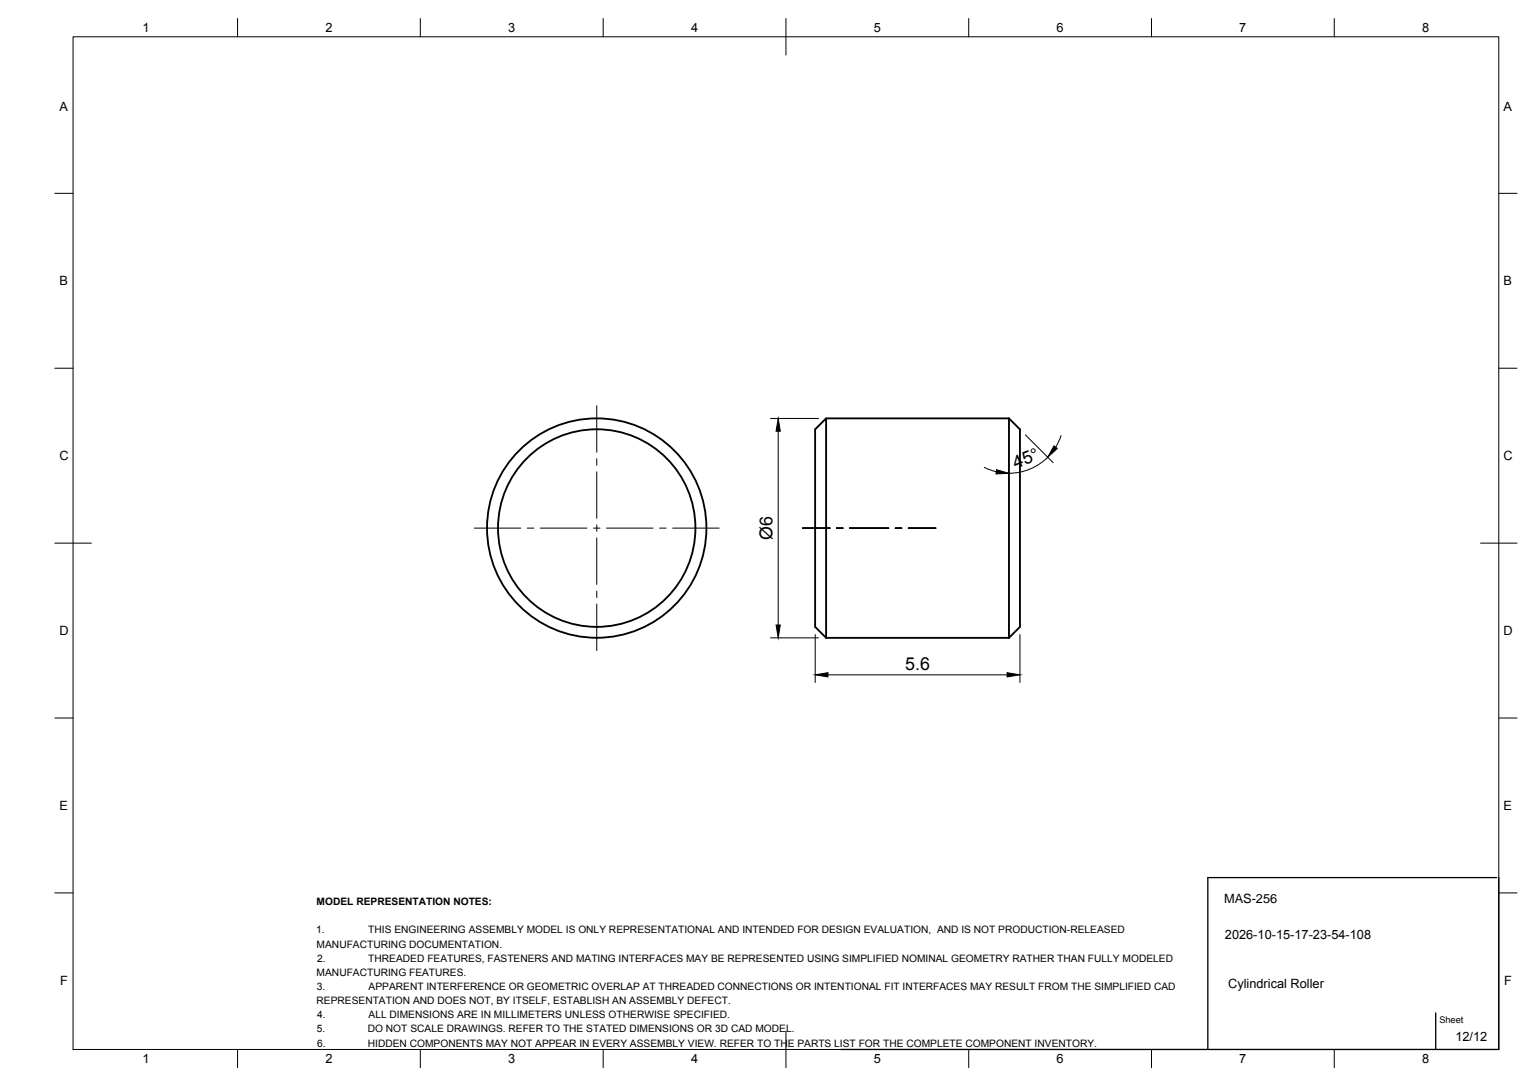
ISO-10303-21;
HEADER;
/* Generated by software containing ST-Developer
 * from STEP Tools, Inc. (www.steptools.com) 
 */

FILE_DESCRIPTION(
/* description */ (''),
/* implementation_level */ '2;1');

FILE_NAME(
/* name */ 'Cylindrical Roller.step',
/* time_stamp */ '2026-10-14T18:40:07-07:00',
/* author */ (''),
/* organization */ (''),
/* preprocessor_version */ 'ST-DEVELOPER v20.2',
/* originating_system */ 'Autodesk Translation Framework v15.15.0.0',
/* authorisation */ '');

FILE_SCHEMA (('AUTOMOTIVE_DESIGN { 1 0 10303 214 3 1 1 }'));
ENDSEC;

DATA;
#10=MECHANICAL_DESIGN_GEOMETRIC_PRESENTATION_REPRESENTATION('',(#836),#81040);
#816=SHAPE_REPRESENTATION_RELATIONSHIP('SRR','None',#81135,#826);
#826=ADVANCED_BREP_SHAPE_REPRESENTATION('',(#846),#81035);
#836=STYLED_ITEM('',(#81194),#846);
#846=MANIFOLD_SOLID_BREP('Body1',#15089);
#990=CYLINDRICAL_SURFACE('',#16080,3.);
#1428=PLANE('',#16076);
#1429=PLANE('',#16084);
#2049=FACE_OUTER_BOUND('',#2915,.T.);
#2050=FACE_OUTER_BOUND('',#2916,.T.);
#2051=FACE_OUTER_BOUND('',#2917,.T.);
#2052=FACE_OUTER_BOUND('',#2918,.T.);
#2053=FACE_OUTER_BOUND('',#2919,.T.);
#2915=EDGE_LOOP('',(#12168));
#2916=EDGE_LOOP('',(#12169,#12170,#12171,#12172));
#2917=EDGE_LOOP('',(#12173,#12174,#12175,#12176));
#2918=EDGE_LOOP('',(#12177,#12178,#12179,#12180));
#2919=EDGE_LOOP('',(#12181));
#3986=LINE('',#23024,#5098);
#3987=LINE('',#23028,#5099);
#3988=LINE('',#23031,#5100);
#5098=VECTOR('',#19136,2.85);
#5099=VECTOR('',#19141,3.);
#5100=VECTOR('',#19144,2.85);
#5837=CIRCLE('',#16077,2.7);
#5838=CIRCLE('',#16079,3.);
#5839=CIRCLE('',#16081,3.);
#5840=CIRCLE('',#16083,2.7);
#6804=VERTEX_POINT('',#23019);
#6805=VERTEX_POINT('',#23022);
#6806=VERTEX_POINT('',#23026);
#6807=VERTEX_POINT('',#23030);
#8747=EDGE_CURVE('',#6804,#6804,#5837,.T.);
#8748=EDGE_CURVE('',#6805,#6805,#5838,.T.);
#8749=EDGE_CURVE('',#6805,#6804,#3986,.T.);
#8750=EDGE_CURVE('',#6806,#6806,#5839,.T.);
#8751=EDGE_CURVE('',#6806,#6805,#3987,.T.);
#8752=EDGE_CURVE('',#6806,#6807,#3988,.T.);
#8753=EDGE_CURVE('',#6807,#6807,#5840,.T.);
#12168=ORIENTED_EDGE('',*,*,#8747,.F.);
#12169=ORIENTED_EDGE('',*,*,#8748,.F.);
#12170=ORIENTED_EDGE('',*,*,#8749,.T.);
#12171=ORIENTED_EDGE('',*,*,#8747,.T.);
#12172=ORIENTED_EDGE('',*,*,#8749,.F.);
#12173=ORIENTED_EDGE('',*,*,#8750,.F.);
#12174=ORIENTED_EDGE('',*,*,#8751,.T.);
#12175=ORIENTED_EDGE('',*,*,#8748,.T.);
#12176=ORIENTED_EDGE('',*,*,#8751,.F.);
#12177=ORIENTED_EDGE('',*,*,#8750,.T.);
#12178=ORIENTED_EDGE('',*,*,#8752,.T.);
#12179=ORIENTED_EDGE('',*,*,#8753,.F.);
#12180=ORIENTED_EDGE('',*,*,#8752,.F.);
#12181=ORIENTED_EDGE('',*,*,#8753,.T.);
#14325=CONICAL_SURFACE('',#16078,2.85,0.785398163397441);
#14326=CONICAL_SURFACE('',#16082,2.85,0.785398163397434);
#14784=ADVANCED_FACE('',(#2049),#1428,.T.);
#14785=ADVANCED_FACE('',(#2050),#14325,.T.);
#14786=ADVANCED_FACE('',(#2051),#990,.T.);
#14787=ADVANCED_FACE('',(#2052),#14326,.T.);
#14788=ADVANCED_FACE('',(#2053),#1429,.T.);
#15089=CLOSED_SHELL('',(#14784,#14785,#14786,#14787,#14788));
#16075=AXIS2_PLACEMENT_3D('',#23017,#19126,#19127);
#16076=AXIS2_PLACEMENT_3D('',#23018,#19128,#19129);
#16077=AXIS2_PLACEMENT_3D('',#23020,#19130,#19131);
#16078=AXIS2_PLACEMENT_3D('',#23021,#19132,#19133);
#16079=AXIS2_PLACEMENT_3D('',#23023,#19134,#19135);
#16080=AXIS2_PLACEMENT_3D('',#23025,#19137,#19138);
#16081=AXIS2_PLACEMENT_3D('',#23027,#19139,#19140);
#16082=AXIS2_PLACEMENT_3D('',#23029,#19142,#19143);
#16083=AXIS2_PLACEMENT_3D('',#23032,#19145,#19146);
#16084=AXIS2_PLACEMENT_3D('',#23033,#19147,#19148);
#19126=DIRECTION('axis',(0.,0.,1.));
#19127=DIRECTION('refdir',(1.,0.,0.));
#19128=DIRECTION('center_axis',(0.,1.,0.));
#19129=DIRECTION('ref_axis',(0.,0.,1.));
#19130=DIRECTION('center_axis',(0.,-1.,0.));
#19131=DIRECTION('ref_axis',(1.,0.,0.));
#19132=DIRECTION('center_axis',(0.,-1.,0.));
#19133=DIRECTION('ref_axis',(1.,0.,0.));
#19134=DIRECTION('center_axis',(0.,-1.,0.));
#19135=DIRECTION('ref_axis',(1.,0.,0.));
#19136=DIRECTION('',(0.707106781186542,0.707106781186553,8.65956056235487E-17));
#19137=DIRECTION('center_axis',(0.,-1.,0.));
#19138=DIRECTION('ref_axis',(1.,0.,0.));
#19139=DIRECTION('center_axis',(0.,-1.,0.));
#19140=DIRECTION('ref_axis',(1.,0.,0.));
#19141=DIRECTION('',(0.,1.,0.));
#19142=DIRECTION('center_axis',(0.,1.,0.));
#19143=DIRECTION('ref_axis',(1.,0.,0.));
#19144=DIRECTION('',(0.707106781186537,-0.707106781186558,-8.65956056235481E-17));
#19145=DIRECTION('center_axis',(0.,-1.,0.));
#19146=DIRECTION('ref_axis',(1.,0.,0.));
#19147=DIRECTION('center_axis',(0.,-1.,0.));
#19148=DIRECTION('ref_axis',(0.,0.,-1.));
#23017=CARTESIAN_POINT('',(0.,0.,0.));
#23018=CARTESIAN_POINT('Origin',(47.7,23.8,32.));
#23019=CARTESIAN_POINT('',(42.3,23.8,32.));
#23020=CARTESIAN_POINT('Origin',(45.,23.8,32.));
#23021=CARTESIAN_POINT('Origin',(45.,23.65,32.));
#23022=CARTESIAN_POINT('',(42.,23.5,32.));
#23023=CARTESIAN_POINT('Origin',(45.,23.5,32.));
#23024=CARTESIAN_POINT('',(42.15,23.65,32.));
#23025=CARTESIAN_POINT('Origin',(45.,21.,32.));
#23026=CARTESIAN_POINT('',(42.,18.5,32.));
#23027=CARTESIAN_POINT('Origin',(45.,18.5,32.));
#23028=CARTESIAN_POINT('',(42.,21.,32.));
#23029=CARTESIAN_POINT('Origin',(45.,18.35,32.));
#23030=CARTESIAN_POINT('',(42.3,18.2,32.));
#23031=CARTESIAN_POINT('',(42.15,18.35,32.));
#23032=CARTESIAN_POINT('Origin',(45.,18.2,32.));
#23033=CARTESIAN_POINT('Origin',(45.,18.2,32.));
#81023=UNCERTAINTY_MEASURE_WITH_UNIT(LENGTH_MEASURE(0.01),#81041,
'DISTANCE_ACCURACY_VALUE',
'Maximum model space distance between geometric entities at asserted c
onnectivities');
#81028=UNCERTAINTY_MEASURE_WITH_UNIT(LENGTH_MEASURE(0.01),#81041,
'DISTANCE_ACCURACY_VALUE',
'Maximum model space distance between geometric entities at asserted c
onnectivities');
#81035=(
GEOMETRIC_REPRESENTATION_CONTEXT(3)
GLOBAL_UNCERTAINTY_ASSIGNED_CONTEXT((#81023))
GLOBAL_UNIT_ASSIGNED_CONTEXT((#81041,#81043,#81044))
REPRESENTATION_CONTEXT('','3D')
);
#81040=(
GEOMETRIC_REPRESENTATION_CONTEXT(3)
GLOBAL_UNCERTAINTY_ASSIGNED_CONTEXT((#81028))
GLOBAL_UNIT_ASSIGNED_CONTEXT((#81041,#81043,#81044))
REPRESENTATION_CONTEXT('','3D')
);
#81041=(
LENGTH_UNIT()
NAMED_UNIT(*)
SI_UNIT(.MILLI.,.METRE.)
);
#81043=(
NAMED_UNIT(*)
PLANE_ANGLE_UNIT()
SI_UNIT($,.RADIAN.)
);
#81044=(
NAMED_UNIT(*)
SI_UNIT($,.STERADIAN.)
SOLID_ANGLE_UNIT()
);
#81051=SHAPE_DEFINITION_REPRESENTATION(#81062,#81135);
#81062=PRODUCT_DEFINITION_SHAPE('',$,#81147);
#81135=SHAPE_REPRESENTATION('',(#16075),#81035);
#81140=PRODUCT_DEFINITION_CONTEXT('part definition',#81175,'design');
#81147=PRODUCT_DEFINITION('Cylindrical Roller','Cylindrical Roller',#81158,
#81140);
#81158=PRODUCT_DEFINITION_FORMATION('',$,#81183);
#81175=APPLICATION_CONTEXT(
'Core Data for Automotive Mechanical Design Process');
#81176=PRODUCT_CONTEXT('part definition',#81175,'mechanical');
#81183=PRODUCT('Cylindrical Roller','Cylindrical Roller',$,(#81176));
#81194=PRESENTATION_STYLE_ASSIGNMENT((#81205));
#81205=SURFACE_STYLE_USAGE(.BOTH.,#81216);
#81216=SURFACE_SIDE_STYLE('',(#81227));
#81227=SURFACE_STYLE_FILL_AREA(#81238);
#81238=FILL_AREA_STYLE('Opaque(238,239,241)',(#81249));
#81249=FILL_AREA_STYLE_COLOUR('Opaque(238,239,241)',#81260);
#81260=COLOUR_RGB('Opaque(238,239,241)', 0.08235294, 0.09019608, 0.10196078);
ENDSEC;
END-ISO-10303-21;
